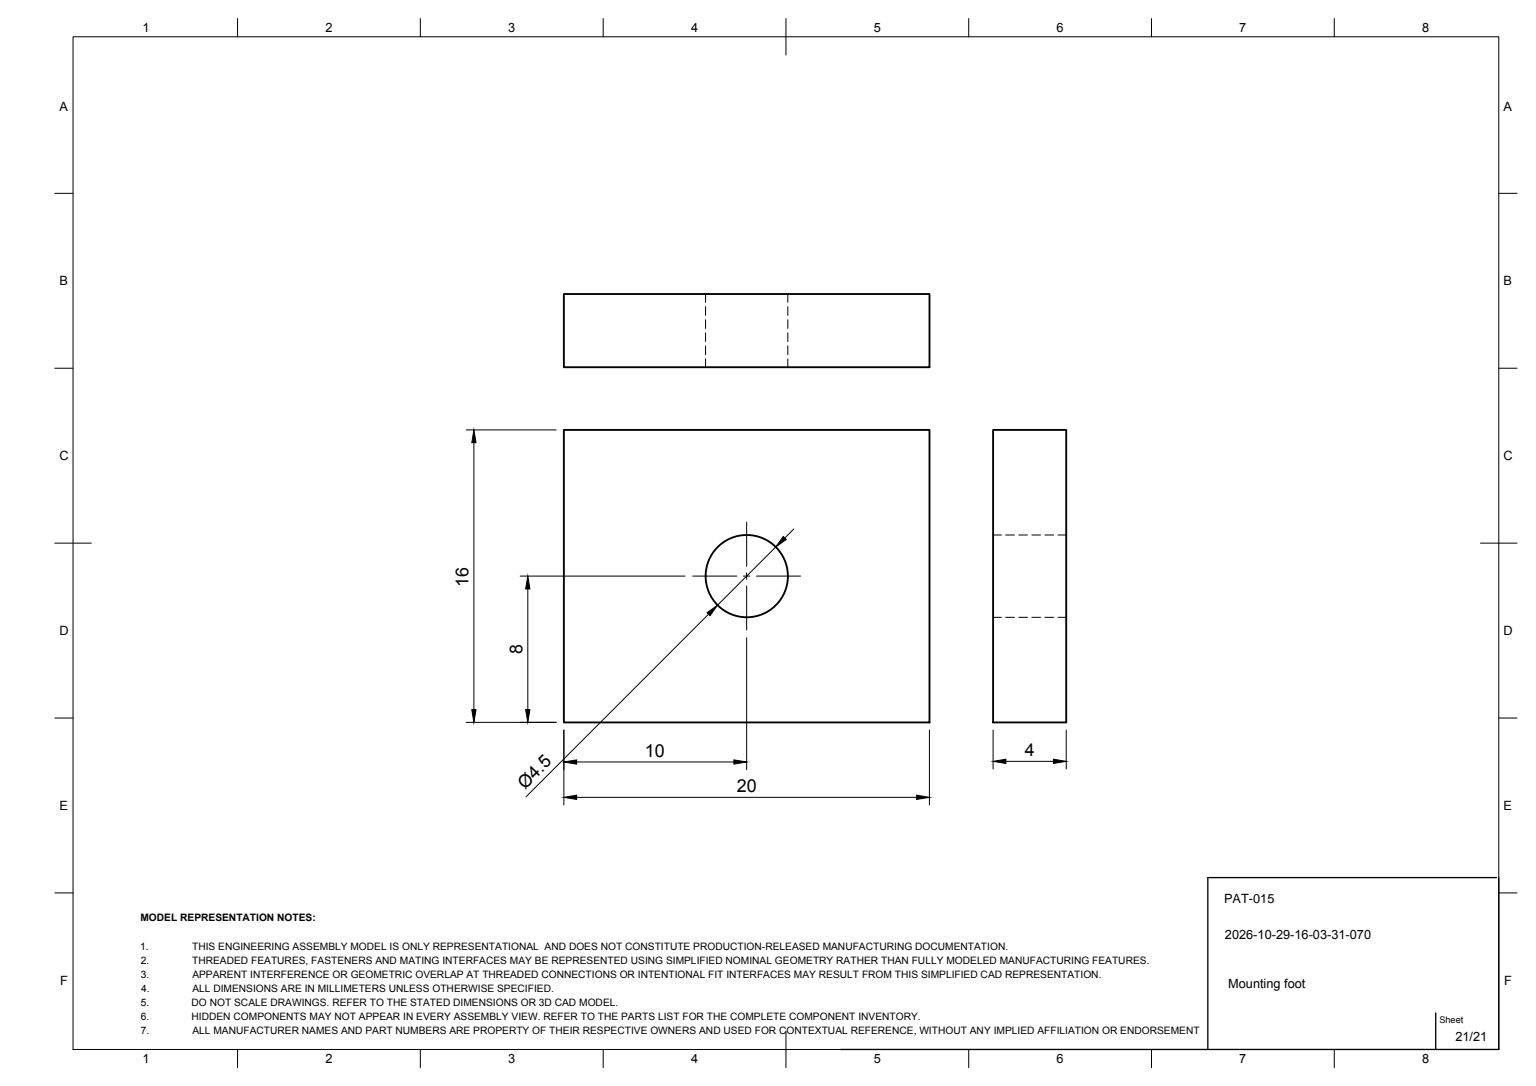
ISO-10303-21;
HEADER;
/* Generated by software containing ST-Developer
 * from STEP Tools, Inc. (www.steptools.com) 
 */

FILE_DESCRIPTION(
/* description */ ('PAT-015'),
/* implementation_level */ '2;1');

FILE_NAME(
/* name */ 'Mounting foot.step',
/* time_stamp */ '2026-10-29T16:03:43-07:00',
/* author */ (''),
/* organization */ (''),
/* preprocessor_version */ 'ST-DEVELOPER v20.2',
/* originating_system */ 'Autodesk Translation Framework v15.17.0.0',
/* authorisation */ '');

FILE_SCHEMA (('AUTOMOTIVE_DESIGN { 1 0 10303 214 3 1 1 }'));
ENDSEC;

DATA;
#10=MECHANICAL_DESIGN_GEOMETRIC_PRESENTATION_REPRESENTATION('',(#253),#10266);
#205=SHAPE_REPRESENTATION_RELATIONSHIP('SRR','None',#10376,#228);
#228=ADVANCED_BREP_SHAPE_REPRESENTATION('',(#277),#10264);
#253=STYLED_ITEM('',(#10540),#277);
#277=MANIFOLD_SOLID_BREP('Body1',#4713);
#417=FACE_BOUND('',#1244,.T.);
#418=FACE_BOUND('',#1246,.T.);
#554=PLANE('',#5489);
#555=PLANE('',#5490);
#556=PLANE('',#5491);
#557=PLANE('',#5492);
#558=PLANE('',#5493);
#559=PLANE('',#5494);
#830=FACE_OUTER_BOUND('',#1238,.T.);
#831=FACE_OUTER_BOUND('',#1239,.T.);
#832=FACE_OUTER_BOUND('',#1240,.T.);
#833=FACE_OUTER_BOUND('',#1241,.T.);
#834=FACE_OUTER_BOUND('',#1242,.T.);
#835=FACE_OUTER_BOUND('',#1243,.T.);
#836=FACE_OUTER_BOUND('',#1245,.T.);
#1238=EDGE_LOOP('',(#4197,#4198,#4199,#4200));
#1239=EDGE_LOOP('',(#4201,#4202,#4203,#4204));
#1240=EDGE_LOOP('',(#4205,#4206,#4207,#4208));
#1241=EDGE_LOOP('',(#4209,#4210,#4211,#4212));
#1242=EDGE_LOOP('',(#4213,#4214,#4215,#4216));
#1243=EDGE_LOOP('',(#4217,#4218,#4219,#4220));
#1244=EDGE_LOOP('',(#4221));
#1245=EDGE_LOOP('',(#4222,#4223,#4224,#4225));
#1246=EDGE_LOOP('',(#4226));
#1566=LINE('',#10084,#1846);
#1567=LINE('',#10089,#1847);
#1568=LINE('',#10091,#1848);
#1569=LINE('',#10093,#1849);
#1570=LINE('',#10094,#1850);
#1571=LINE('',#10097,#1851);
#1572=LINE('',#10099,#1852);
#1573=LINE('',#10100,#1853);
#1574=LINE('',#10103,#1854);
#1575=LINE('',#10105,#1855);
#1576=LINE('',#10106,#1856);
#1577=LINE('',#10108,#1857);
#1578=LINE('',#10109,#1858);
#1846=VECTOR('',#6835,0.225);
#1847=VECTOR('',#6840,1.);
#1848=VECTOR('',#6841,1.);
#1849=VECTOR('',#6842,1.);
#1850=VECTOR('',#6843,1.);
#1851=VECTOR('',#6846,1.);
#1852=VECTOR('',#6847,1.);
#1853=VECTOR('',#6848,1.);
#1854=VECTOR('',#6851,1.);
#1855=VECTOR('',#6852,1.);
#1856=VECTOR('',#6853,1.);
#1857=VECTOR('',#6856,1.);
#1858=VECTOR('',#6857,1.);
#2104=CIRCLE('',#5487,0.225);
#2105=CIRCLE('',#5488,0.225);
#2476=VERTEX_POINT('',#10081);
#2477=VERTEX_POINT('',#10083);
#2478=VERTEX_POINT('',#10087);
#2479=VERTEX_POINT('',#10088);
#2480=VERTEX_POINT('',#10090);
#2481=VERTEX_POINT('',#10092);
#2482=VERTEX_POINT('',#10096);
#2483=VERTEX_POINT('',#10098);
#2484=VERTEX_POINT('',#10102);
#2485=VERTEX_POINT('',#10104);
#3054=EDGE_CURVE('',#2476,#2476,#2104,.T.);
#3055=EDGE_CURVE('',#2476,#2477,#1566,.T.);
#3056=EDGE_CURVE('',#2477,#2477,#2105,.T.);
#3057=EDGE_CURVE('',#2478,#2479,#1567,.T.);
#3058=EDGE_CURVE('',#2479,#2480,#1568,.T.);
#3059=EDGE_CURVE('',#2481,#2480,#1569,.T.);
#3060=EDGE_CURVE('',#2478,#2481,#1570,.T.);
#3061=EDGE_CURVE('',#2482,#2478,#1571,.T.);
#3062=EDGE_CURVE('',#2483,#2481,#1572,.T.);
#3063=EDGE_CURVE('',#2482,#2483,#1573,.T.);
#3064=EDGE_CURVE('',#2484,#2482,#1574,.T.);
#3065=EDGE_CURVE('',#2485,#2483,#1575,.T.);
#3066=EDGE_CURVE('',#2484,#2485,#1576,.T.);
#3067=EDGE_CURVE('',#2479,#2484,#1577,.T.);
#3068=EDGE_CURVE('',#2480,#2485,#1578,.T.);
#4197=ORIENTED_EDGE('',*,*,#3054,.F.);
#4198=ORIENTED_EDGE('',*,*,#3055,.T.);
#4199=ORIENTED_EDGE('',*,*,#3056,.F.);
#4200=ORIENTED_EDGE('',*,*,#3055,.F.);
#4201=ORIENTED_EDGE('',*,*,#3057,.T.);
#4202=ORIENTED_EDGE('',*,*,#3058,.T.);
#4203=ORIENTED_EDGE('',*,*,#3059,.F.);
#4204=ORIENTED_EDGE('',*,*,#3060,.F.);
#4205=ORIENTED_EDGE('',*,*,#3061,.T.);
#4206=ORIENTED_EDGE('',*,*,#3060,.T.);
#4207=ORIENTED_EDGE('',*,*,#3062,.F.);
#4208=ORIENTED_EDGE('',*,*,#3063,.F.);
#4209=ORIENTED_EDGE('',*,*,#3064,.T.);
#4210=ORIENTED_EDGE('',*,*,#3063,.T.);
#4211=ORIENTED_EDGE('',*,*,#3065,.F.);
#4212=ORIENTED_EDGE('',*,*,#3066,.F.);
#4213=ORIENTED_EDGE('',*,*,#3067,.T.);
#4214=ORIENTED_EDGE('',*,*,#3066,.T.);
#4215=ORIENTED_EDGE('',*,*,#3068,.F.);
#4216=ORIENTED_EDGE('',*,*,#3058,.F.);
#4217=ORIENTED_EDGE('',*,*,#3068,.T.);
#4218=ORIENTED_EDGE('',*,*,#3065,.T.);
#4219=ORIENTED_EDGE('',*,*,#3062,.T.);
#4220=ORIENTED_EDGE('',*,*,#3059,.T.);
#4221=ORIENTED_EDGE('',*,*,#3056,.T.);
#4222=ORIENTED_EDGE('',*,*,#3067,.F.);
#4223=ORIENTED_EDGE('',*,*,#3057,.F.);
#4224=ORIENTED_EDGE('',*,*,#3061,.F.);
#4225=ORIENTED_EDGE('',*,*,#3064,.F.);
#4226=ORIENTED_EDGE('',*,*,#3054,.T.);
#4403=CYLINDRICAL_SURFACE('',#5486,0.225);
#4665=ADVANCED_FACE('',(#830),#4403,.F.);
#4666=ADVANCED_FACE('',(#831),#554,.T.);
#4667=ADVANCED_FACE('',(#832),#555,.T.);
#4668=ADVANCED_FACE('',(#833),#556,.T.);
#4669=ADVANCED_FACE('',(#834),#557,.T.);
#4670=ADVANCED_FACE('',(#835,#417),#558,.T.);
#4671=ADVANCED_FACE('',(#836,#418),#559,.F.);
#4713=CLOSED_SHELL('',(#4665,#4666,#4667,#4668,#4669,#4670,#4671));
#5485=AXIS2_PLACEMENT_3D('',#10079,#6829,#6830);
#5486=AXIS2_PLACEMENT_3D('',#10080,#6831,#6832);
#5487=AXIS2_PLACEMENT_3D('',#10082,#6833,#6834);
#5488=AXIS2_PLACEMENT_3D('',#10085,#6836,#6837);
#5489=AXIS2_PLACEMENT_3D('',#10086,#6838,#6839);
#5490=AXIS2_PLACEMENT_3D('',#10095,#6844,#6845);
#5491=AXIS2_PLACEMENT_3D('',#10101,#6849,#6850);
#5492=AXIS2_PLACEMENT_3D('',#10107,#6854,#6855);
#5493=AXIS2_PLACEMENT_3D('',#10110,#6858,#6859);
#5494=AXIS2_PLACEMENT_3D('',#10111,#6860,#6861);
#6829=DIRECTION('axis',(0.,0.,1.));
#6830=DIRECTION('refdir',(1.,0.,0.));
#6831=DIRECTION('center_axis',(0.,0.,1.));
#6832=DIRECTION('ref_axis',(1.,0.,0.));
#6833=DIRECTION('center_axis',(0.,0.,1.));
#6834=DIRECTION('ref_axis',(1.,0.,0.));
#6835=DIRECTION('',(0.,0.,1.));
#6836=DIRECTION('center_axis',(0.,0.,-1.));
#6837=DIRECTION('ref_axis',(1.,0.,0.));
#6838=DIRECTION('center_axis',(0.,1.,0.));
#6839=DIRECTION('ref_axis',(-1.,0.,0.));
#6840=DIRECTION('',(-1.,0.,0.));
#6841=DIRECTION('',(0.,0.,1.));
#6842=DIRECTION('',(-1.,0.,0.));
#6843=DIRECTION('',(0.,0.,1.));
#6844=DIRECTION('center_axis',(1.,0.,0.));
#6845=DIRECTION('ref_axis',(0.,1.,0.));
#6846=DIRECTION('',(0.,1.,0.));
#6847=DIRECTION('',(0.,1.,0.));
#6848=DIRECTION('',(0.,0.,1.));
#6849=DIRECTION('center_axis',(0.,-1.,0.));
#6850=DIRECTION('ref_axis',(1.,0.,0.));
#6851=DIRECTION('',(1.,0.,0.));
#6852=DIRECTION('',(1.,0.,0.));
#6853=DIRECTION('',(0.,0.,1.));
#6854=DIRECTION('center_axis',(-1.,0.,0.));
#6855=DIRECTION('ref_axis',(0.,-1.,0.));
#6856=DIRECTION('',(0.,-1.,0.));
#6857=DIRECTION('',(0.,-1.,0.));
#6858=DIRECTION('center_axis',(0.,0.,1.));
#6859=DIRECTION('ref_axis',(1.,0.,0.));
#6860=DIRECTION('center_axis',(0.,0.,1.));
#6861=DIRECTION('ref_axis',(1.,0.,0.));
#10079=CARTESIAN_POINT('',(0.,0.,0.));
#10080=CARTESIAN_POINT('Origin',(0.,-3.,0.5));
#10081=CARTESIAN_POINT('',(-0.225,-3.,0.6));
#10082=CARTESIAN_POINT('Origin',(0.,-3.,0.6));
#10083=CARTESIAN_POINT('',(-0.225,-3.,1.));
#10084=CARTESIAN_POINT('',(-0.225,-3.,0.5));
#10085=CARTESIAN_POINT('Origin',(0.,-3.,1.));
#10086=CARTESIAN_POINT('Origin',(1.,-2.2,0.6));
#10087=CARTESIAN_POINT('',(1.,-2.2,0.6));
#10088=CARTESIAN_POINT('',(-1.,-2.2,0.6));
#10089=CARTESIAN_POINT('',(1.,-2.2,0.6));
#10090=CARTESIAN_POINT('',(-1.,-2.2,1.));
#10091=CARTESIAN_POINT('',(-1.,-2.2,0.6));
#10092=CARTESIAN_POINT('',(1.,-2.2,1.));
#10093=CARTESIAN_POINT('',(1.,-2.2,1.));
#10094=CARTESIAN_POINT('',(1.,-2.2,0.6));
#10095=CARTESIAN_POINT('Origin',(1.,-3.8,0.6));
#10096=CARTESIAN_POINT('',(1.,-3.8,0.6));
#10097=CARTESIAN_POINT('',(1.,-3.8,0.6));
#10098=CARTESIAN_POINT('',(1.,-3.8,1.));
#10099=CARTESIAN_POINT('',(1.,-3.8,1.));
#10100=CARTESIAN_POINT('',(1.,-3.8,0.6));
#10101=CARTESIAN_POINT('Origin',(-1.,-3.8,0.6));
#10102=CARTESIAN_POINT('',(-1.,-3.8,0.6));
#10103=CARTESIAN_POINT('',(-1.,-3.8,0.6));
#10104=CARTESIAN_POINT('',(-1.,-3.8,1.));
#10105=CARTESIAN_POINT('',(-1.,-3.8,1.));
#10106=CARTESIAN_POINT('',(-1.,-3.8,0.6));
#10107=CARTESIAN_POINT('Origin',(-1.,-2.2,0.6));
#10108=CARTESIAN_POINT('',(-1.,-2.2,0.6));
#10109=CARTESIAN_POINT('',(-1.,-2.2,1.));
#10110=CARTESIAN_POINT('Origin',(0.,-3.,1.));
#10111=CARTESIAN_POINT('Origin',(0.,-3.,0.6));
#10239=UNCERTAINTY_MEASURE_WITH_UNIT(LENGTH_MEASURE(0.001),#10267,
'DISTANCE_ACCURACY_VALUE',
'Maximum model space distance between geometric entities at asserted c
onnectivities');
#10241=UNCERTAINTY_MEASURE_WITH_UNIT(LENGTH_MEASURE(0.001),#10267,
'DISTANCE_ACCURACY_VALUE',
'Maximum model space distance between geometric entities at asserted c
onnectivities');
#10264=(
GEOMETRIC_REPRESENTATION_CONTEXT(3)
GLOBAL_UNCERTAINTY_ASSIGNED_CONTEXT((#10239))
GLOBAL_UNIT_ASSIGNED_CONTEXT((#10267,#10269,#10270))
REPRESENTATION_CONTEXT('','3D')
);
#10266=(
GEOMETRIC_REPRESENTATION_CONTEXT(3)
GLOBAL_UNCERTAINTY_ASSIGNED_CONTEXT((#10241))
GLOBAL_UNIT_ASSIGNED_CONTEXT((#10267,#10269,#10270))
REPRESENTATION_CONTEXT('','3D')
);
#10267=(
LENGTH_UNIT()
NAMED_UNIT(*)
SI_UNIT(.CENTI.,.METRE.)
);
#10269=(
NAMED_UNIT(*)
PLANE_ANGLE_UNIT()
SI_UNIT($,.RADIAN.)
);
#10270=(
NAMED_UNIT(*)
SI_UNIT($,.STERADIAN.)
SOLID_ANGLE_UNIT()
);
#10293=SHAPE_DEFINITION_REPRESENTATION(#10317,#10376);
#10317=PRODUCT_DEFINITION_SHAPE('',$,#10401);
#10376=SHAPE_REPRESENTATION('',(#5485),#10264);
#10378=PRODUCT_DEFINITION_CONTEXT('part definition',#10452,'design');
#10401=PRODUCT_DEFINITION('Mounting foot','Mounting foot',#10425,
#10378);
#10425=PRODUCT_DEFINITION_FORMATION('',$,#10476);
#10452=APPLICATION_CONTEXT(
'Core Data for Automotive Mechanical Design Process');
#10453=PRODUCT_CONTEXT('part definition',#10452,'mechanical');
#10476=PRODUCT('Mounting foot','Mounting foot',
'Mounting foot',(#10453));
#10534=COLOUR_RGB('Sky Blue',0.24,0.69,0.87);
#10535=FILL_AREA_STYLE_COLOUR('',#10534);
#10536=FILL_AREA_STYLE('',(#10535));
#10537=SURFACE_STYLE_FILL_AREA(#10536);
#10538=SURFACE_SIDE_STYLE('',(#10537));
#10539=SURFACE_STYLE_USAGE(.BOTH.,#10538);
#10540=PRESENTATION_STYLE_ASSIGNMENT((#10539));
ENDSEC;
END-ISO-10303-21;
